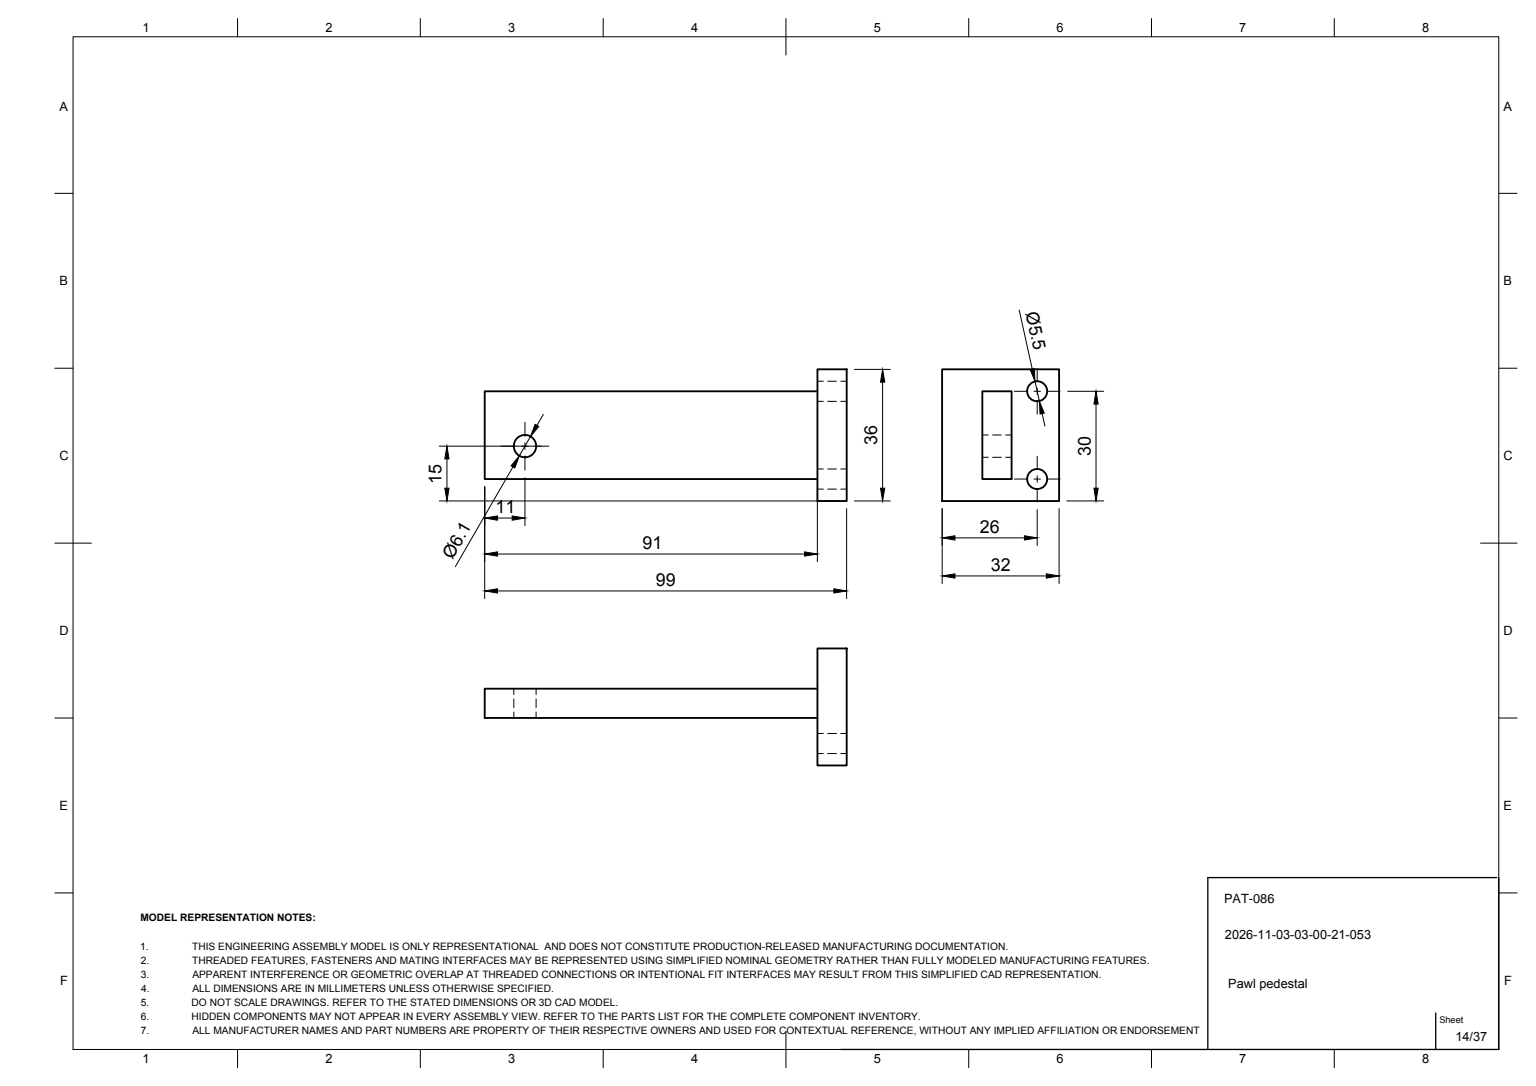
ISO-10303-21;
HEADER;
/* Generated by software containing ST-Developer
 * from STEP Tools, Inc. (www.steptools.com) 
 */

FILE_DESCRIPTION(
/* description */ ('Ratchet and pawl hand winch drum'),
/* implementation_level */ '2;1');

FILE_NAME(
/* name */ 'Pawl pedestal.step',
/* time_stamp */ '2026-10-27T12:42:58-07:00',
/* author */ (''),
/* organization */ (''),
/* preprocessor_version */ 'ST-DEVELOPER v20.2',
/* originating_system */ 'Autodesk Translation Framework v15.17.0.0',
/* authorisation */ '');

FILE_SCHEMA (('AUTOMOTIVE_DESIGN { 1 0 10303 214 3 1 1 }'));
ENDSEC;

DATA;
#10=MECHANICAL_DESIGN_GEOMETRIC_PRESENTATION_REPRESENTATION('',(#398),#11801);
#330=SHAPE_REPRESENTATION_RELATIONSHIP('SRR','None',#11956,#364);
#364=ADVANCED_BREP_SHAPE_REPRESENTATION('',(#433),#11773);
#398=STYLED_ITEM('',(#12206),#433);
#433=MANIFOLD_SOLID_BREP('Body1',#6275);
#516=FACE_BOUND('',#1344,.T.);
#517=FACE_BOUND('',#1345,.T.);
#518=FACE_BOUND('',#1346,.T.);
#519=FACE_BOUND('',#1352,.T.);
#520=FACE_BOUND('',#1355,.T.);
#521=FACE_BOUND('',#1359,.T.);
#522=FACE_BOUND('',#1360,.T.);
#647=PLANE('',#6860);
#648=PLANE('',#6861);
#649=PLANE('',#6862);
#650=PLANE('',#6863);
#651=PLANE('',#6864);
#652=PLANE('',#6865);
#653=PLANE('',#6866);
#654=PLANE('',#6867);
#655=PLANE('',#6868);
#656=PLANE('',#6869);
#657=PLANE('',#6870);
#924=FACE_OUTER_BOUND('',#1340,.T.);
#925=FACE_OUTER_BOUND('',#1341,.T.);
#926=FACE_OUTER_BOUND('',#1342,.T.);
#927=FACE_OUTER_BOUND('',#1343,.T.);
#928=FACE_OUTER_BOUND('',#1347,.T.);
#929=FACE_OUTER_BOUND('',#1348,.T.);
#930=FACE_OUTER_BOUND('',#1349,.T.);
#931=FACE_OUTER_BOUND('',#1350,.T.);
#932=FACE_OUTER_BOUND('',#1351,.T.);
#933=FACE_OUTER_BOUND('',#1353,.T.);
#934=FACE_OUTER_BOUND('',#1354,.T.);
#935=FACE_OUTER_BOUND('',#1356,.T.);
#936=FACE_OUTER_BOUND('',#1357,.T.);
#937=FACE_OUTER_BOUND('',#1358,.T.);
#1340=EDGE_LOOP('',(#4595,#4596,#4597,#4598));
#1341=EDGE_LOOP('',(#4599,#4600,#4601,#4602));
#1342=EDGE_LOOP('',(#4603,#4604,#4605,#4606));
#1343=EDGE_LOOP('',(#4607,#4608,#4609,#4610));
#1344=EDGE_LOOP('',(#4611));
#1345=EDGE_LOOP('',(#4612));
#1346=EDGE_LOOP('',(#4613,#4614,#4615,#4616));
#1347=EDGE_LOOP('',(#4617,#4618,#4619,#4620));
#1348=EDGE_LOOP('',(#4621,#4622,#4623,#4624));
#1349=EDGE_LOOP('',(#4625,#4626,#4627,#4628));
#1350=EDGE_LOOP('',(#4629,#4630,#4631,#4632));
#1351=EDGE_LOOP('',(#4633,#4634,#4635,#4636));
#1352=EDGE_LOOP('',(#4637));
#1353=EDGE_LOOP('',(#4638,#4639,#4640,#4641));
#1354=EDGE_LOOP('',(#4642,#4643,#4644,#4645));
#1355=EDGE_LOOP('',(#4646));
#1356=EDGE_LOOP('',(#4647,#4648,#4649,#4650));
#1357=EDGE_LOOP('',(#4651,#4652,#4653,#4654));
#1358=EDGE_LOOP('',(#4655,#4656,#4657,#4658));
#1359=EDGE_LOOP('',(#4659));
#1360=EDGE_LOOP('',(#4660));
#1795=LINE('',#9617,#2306);
#1796=LINE('',#9623,#2307);
#1797=LINE('',#9629,#2308);
#1798=LINE('',#9634,#2309);
#1799=LINE('',#9636,#2310);
#1800=LINE('',#9638,#2311);
#1801=LINE('',#9639,#2312);
#1802=LINE('',#9642,#2313);
#1803=LINE('',#9644,#2314);
#1804=LINE('',#9646,#2315);
#1805=LINE('',#9647,#2316);
#1806=LINE('',#9650,#2317);
#1807=LINE('',#9652,#2318);
#1808=LINE('',#9653,#2319);
#1809=LINE('',#9656,#2320);
#1810=LINE('',#9658,#2321);
#1811=LINE('',#9659,#2322);
#1812=LINE('',#9661,#2323);
#1813=LINE('',#9663,#2324);
#1814=LINE('',#9666,#2325);
#1815=LINE('',#9668,#2326);
#1816=LINE('',#9669,#2327);
#1817=LINE('',#9672,#2328);
#1818=LINE('',#9673,#2329);
#1819=LINE('',#9676,#2330);
#1820=LINE('',#9677,#2331);
#1821=LINE('',#9679,#2332);
#2306=VECTOR('',#7804,0.275);
#2307=VECTOR('',#7811,0.275);
#2308=VECTOR('',#7818,0.305);
#2309=VECTOR('',#7823,1.);
#2310=VECTOR('',#7824,1.);
#2311=VECTOR('',#7825,1.);
#2312=VECTOR('',#7826,1.);
#2313=VECTOR('',#7827,1.);
#2314=VECTOR('',#7828,1.);
#2315=VECTOR('',#7829,1.);
#2316=VECTOR('',#7830,1.);
#2317=VECTOR('',#7833,1.);
#2318=VECTOR('',#7834,1.);
#2319=VECTOR('',#7835,1.);
#2320=VECTOR('',#7838,1.);
#2321=VECTOR('',#7839,1.);
#2322=VECTOR('',#7840,1.);
#2323=VECTOR('',#7843,1.);
#2324=VECTOR('',#7846,1.);
#2325=VECTOR('',#7849,1.);
#2326=VECTOR('',#7850,1.);
#2327=VECTOR('',#7851,1.);
#2328=VECTOR('',#7854,1.);
#2329=VECTOR('',#7855,1.);
#2330=VECTOR('',#7858,1.);
#2331=VECTOR('',#7859,1.);
#2332=VECTOR('',#7862,1.);
#2795=CIRCLE('',#6852,0.275);
#2796=CIRCLE('',#6853,0.275);
#2797=CIRCLE('',#6855,0.275);
#2798=CIRCLE('',#6856,0.275);
#2799=CIRCLE('',#6858,0.305);
#2800=CIRCLE('',#6859,0.305);
#3058=VERTEX_POINT('',#9614);
#3059=VERTEX_POINT('',#9616);
#3060=VERTEX_POINT('',#9620);
#3061=VERTEX_POINT('',#9622);
#3062=VERTEX_POINT('',#9626);
#3063=VERTEX_POINT('',#9628);
#3064=VERTEX_POINT('',#9632);
#3065=VERTEX_POINT('',#9633);
#3066=VERTEX_POINT('',#9635);
#3067=VERTEX_POINT('',#9637);
#3068=VERTEX_POINT('',#9640);
#3069=VERTEX_POINT('',#9641);
#3070=VERTEX_POINT('',#9643);
#3071=VERTEX_POINT('',#9645);
#3072=VERTEX_POINT('',#9649);
#3073=VERTEX_POINT('',#9651);
#3074=VERTEX_POINT('',#9655);
#3075=VERTEX_POINT('',#9657);
#3076=VERTEX_POINT('',#9665);
#3077=VERTEX_POINT('',#9667);
#3078=VERTEX_POINT('',#9671);
#3079=VERTEX_POINT('',#9675);
#3641=EDGE_CURVE('',#3058,#3058,#2795,.T.);
#3642=EDGE_CURVE('',#3058,#3059,#1795,.T.);
#3643=EDGE_CURVE('',#3059,#3059,#2796,.T.);
#3644=EDGE_CURVE('',#3060,#3060,#2797,.T.);
#3645=EDGE_CURVE('',#3060,#3061,#1796,.T.);
#3646=EDGE_CURVE('',#3061,#3061,#2798,.T.);
#3647=EDGE_CURVE('',#3062,#3062,#2799,.T.);
#3648=EDGE_CURVE('',#3062,#3063,#1797,.T.);
#3649=EDGE_CURVE('',#3063,#3063,#2800,.T.);
#3650=EDGE_CURVE('',#3064,#3065,#1798,.T.);
#3651=EDGE_CURVE('',#3064,#3066,#1799,.T.);
#3652=EDGE_CURVE('',#3067,#3066,#1800,.T.);
#3653=EDGE_CURVE('',#3065,#3067,#1801,.T.);
#3654=EDGE_CURVE('',#3068,#3069,#1802,.T.);
#3655=EDGE_CURVE('',#3070,#3068,#1803,.T.);
#3656=EDGE_CURVE('',#3071,#3070,#1804,.T.);
#3657=EDGE_CURVE('',#3069,#3071,#1805,.T.);
#3658=EDGE_CURVE('',#3065,#3072,#1806,.T.);
#3659=EDGE_CURVE('',#3073,#3067,#1807,.T.);
#3660=EDGE_CURVE('',#3072,#3073,#1808,.T.);
#3661=EDGE_CURVE('',#3074,#3064,#1809,.T.);
#3662=EDGE_CURVE('',#3074,#3075,#1810,.T.);
#3663=EDGE_CURVE('',#3066,#3075,#1811,.T.);
#3664=EDGE_CURVE('',#3075,#3073,#1812,.T.);
#3665=EDGE_CURVE('',#3072,#3074,#1813,.T.);
#3666=EDGE_CURVE('',#3070,#3076,#1814,.T.);
#3667=EDGE_CURVE('',#3077,#3076,#1815,.T.);
#3668=EDGE_CURVE('',#3071,#3077,#1816,.T.);
#3669=EDGE_CURVE('',#3068,#3078,#1817,.T.);
#3670=EDGE_CURVE('',#3076,#3078,#1818,.T.);
#3671=EDGE_CURVE('',#3069,#3079,#1819,.T.);
#3672=EDGE_CURVE('',#3078,#3079,#1820,.T.);
#3673=EDGE_CURVE('',#3079,#3077,#1821,.T.);
#4595=ORIENTED_EDGE('',*,*,#3641,.F.);
#4596=ORIENTED_EDGE('',*,*,#3642,.T.);
#4597=ORIENTED_EDGE('',*,*,#3643,.F.);
#4598=ORIENTED_EDGE('',*,*,#3642,.F.);
#4599=ORIENTED_EDGE('',*,*,#3644,.F.);
#4600=ORIENTED_EDGE('',*,*,#3645,.T.);
#4601=ORIENTED_EDGE('',*,*,#3646,.F.);
#4602=ORIENTED_EDGE('',*,*,#3645,.F.);
#4603=ORIENTED_EDGE('',*,*,#3647,.F.);
#4604=ORIENTED_EDGE('',*,*,#3648,.T.);
#4605=ORIENTED_EDGE('',*,*,#3649,.F.);
#4606=ORIENTED_EDGE('',*,*,#3648,.F.);
#4607=ORIENTED_EDGE('',*,*,#3650,.F.);
#4608=ORIENTED_EDGE('',*,*,#3651,.T.);
#4609=ORIENTED_EDGE('',*,*,#3652,.F.);
#4610=ORIENTED_EDGE('',*,*,#3653,.F.);
#4611=ORIENTED_EDGE('',*,*,#3643,.T.);
#4612=ORIENTED_EDGE('',*,*,#3646,.T.);
#4613=ORIENTED_EDGE('',*,*,#3654,.F.);
#4614=ORIENTED_EDGE('',*,*,#3655,.F.);
#4615=ORIENTED_EDGE('',*,*,#3656,.F.);
#4616=ORIENTED_EDGE('',*,*,#3657,.F.);
#4617=ORIENTED_EDGE('',*,*,#3658,.F.);
#4618=ORIENTED_EDGE('',*,*,#3653,.T.);
#4619=ORIENTED_EDGE('',*,*,#3659,.F.);
#4620=ORIENTED_EDGE('',*,*,#3660,.F.);
#4621=ORIENTED_EDGE('',*,*,#3661,.F.);
#4622=ORIENTED_EDGE('',*,*,#3662,.T.);
#4623=ORIENTED_EDGE('',*,*,#3663,.F.);
#4624=ORIENTED_EDGE('',*,*,#3651,.F.);
#4625=ORIENTED_EDGE('',*,*,#3652,.T.);
#4626=ORIENTED_EDGE('',*,*,#3663,.T.);
#4627=ORIENTED_EDGE('',*,*,#3664,.T.);
#4628=ORIENTED_EDGE('',*,*,#3659,.T.);
#4629=ORIENTED_EDGE('',*,*,#3650,.T.);
#4630=ORIENTED_EDGE('',*,*,#3658,.T.);
#4631=ORIENTED_EDGE('',*,*,#3665,.T.);
#4632=ORIENTED_EDGE('',*,*,#3661,.T.);
#4633=ORIENTED_EDGE('',*,*,#3656,.T.);
#4634=ORIENTED_EDGE('',*,*,#3666,.T.);
#4635=ORIENTED_EDGE('',*,*,#3667,.F.);
#4636=ORIENTED_EDGE('',*,*,#3668,.F.);
#4637=ORIENTED_EDGE('',*,*,#3647,.T.);
#4638=ORIENTED_EDGE('',*,*,#3655,.T.);
#4639=ORIENTED_EDGE('',*,*,#3669,.T.);
#4640=ORIENTED_EDGE('',*,*,#3670,.F.);
#4641=ORIENTED_EDGE('',*,*,#3666,.F.);
#4642=ORIENTED_EDGE('',*,*,#3654,.T.);
#4643=ORIENTED_EDGE('',*,*,#3671,.T.);
#4644=ORIENTED_EDGE('',*,*,#3672,.F.);
#4645=ORIENTED_EDGE('',*,*,#3669,.F.);
#4646=ORIENTED_EDGE('',*,*,#3649,.T.);
#4647=ORIENTED_EDGE('',*,*,#3657,.T.);
#4648=ORIENTED_EDGE('',*,*,#3668,.T.);
#4649=ORIENTED_EDGE('',*,*,#3673,.F.);
#4650=ORIENTED_EDGE('',*,*,#3671,.F.);
#4651=ORIENTED_EDGE('',*,*,#3673,.T.);
#4652=ORIENTED_EDGE('',*,*,#3667,.T.);
#4653=ORIENTED_EDGE('',*,*,#3670,.T.);
#4654=ORIENTED_EDGE('',*,*,#3672,.T.);
#4655=ORIENTED_EDGE('',*,*,#3665,.F.);
#4656=ORIENTED_EDGE('',*,*,#3660,.T.);
#4657=ORIENTED_EDGE('',*,*,#3664,.F.);
#4658=ORIENTED_EDGE('',*,*,#3662,.F.);
#4659=ORIENTED_EDGE('',*,*,#3641,.T.);
#4660=ORIENTED_EDGE('',*,*,#3644,.T.);
#5845=CYLINDRICAL_SURFACE('',#6851,0.275);
#5846=CYLINDRICAL_SURFACE('',#6854,0.275);
#5847=CYLINDRICAL_SURFACE('',#6857,0.305);
#5994=ADVANCED_FACE('',(#924),#5845,.F.);
#5995=ADVANCED_FACE('',(#925),#5846,.F.);
#5996=ADVANCED_FACE('',(#926),#5847,.F.);
#5997=ADVANCED_FACE('',(#927,#516,#517,#518),#647,.T.);
#5998=ADVANCED_FACE('',(#928),#648,.T.);
#5999=ADVANCED_FACE('',(#929),#649,.T.);
#6000=ADVANCED_FACE('',(#930),#650,.T.);
#6001=ADVANCED_FACE('',(#931),#651,.F.);
#6002=ADVANCED_FACE('',(#932,#519),#652,.T.);
#6003=ADVANCED_FACE('',(#933),#653,.T.);
#6004=ADVANCED_FACE('',(#934,#520),#654,.T.);
#6005=ADVANCED_FACE('',(#935),#655,.T.);
#6006=ADVANCED_FACE('',(#936),#656,.T.);
#6007=ADVANCED_FACE('',(#937,#521,#522),#657,.F.);
#6275=CLOSED_SHELL('',(#5994,#5995,#5996,#5997,#5998,#5999,#6000,#6001,
#6002,#6003,#6004,#6005,#6006,#6007));
#6850=AXIS2_PLACEMENT_3D('',#9612,#7798,#7799);
#6851=AXIS2_PLACEMENT_3D('',#9613,#7800,#7801);
#6852=AXIS2_PLACEMENT_3D('',#9615,#7802,#7803);
#6853=AXIS2_PLACEMENT_3D('',#9618,#7805,#7806);
#6854=AXIS2_PLACEMENT_3D('',#9619,#7807,#7808);
#6855=AXIS2_PLACEMENT_3D('',#9621,#7809,#7810);
#6856=AXIS2_PLACEMENT_3D('',#9624,#7812,#7813);
#6857=AXIS2_PLACEMENT_3D('',#9625,#7814,#7815);
#6858=AXIS2_PLACEMENT_3D('',#9627,#7816,#7817);
#6859=AXIS2_PLACEMENT_3D('',#9630,#7819,#7820);
#6860=AXIS2_PLACEMENT_3D('',#9631,#7821,#7822);
#6861=AXIS2_PLACEMENT_3D('',#9648,#7831,#7832);
#6862=AXIS2_PLACEMENT_3D('',#9654,#7836,#7837);
#6863=AXIS2_PLACEMENT_3D('',#9660,#7841,#7842);
#6864=AXIS2_PLACEMENT_3D('',#9662,#7844,#7845);
#6865=AXIS2_PLACEMENT_3D('',#9664,#7847,#7848);
#6866=AXIS2_PLACEMENT_3D('',#9670,#7852,#7853);
#6867=AXIS2_PLACEMENT_3D('',#9674,#7856,#7857);
#6868=AXIS2_PLACEMENT_3D('',#9678,#7860,#7861);
#6869=AXIS2_PLACEMENT_3D('',#9680,#7863,#7864);
#6870=AXIS2_PLACEMENT_3D('',#9681,#7865,#7866);
#7798=DIRECTION('axis',(0.,0.,1.));
#7799=DIRECTION('refdir',(1.,0.,0.));
#7800=DIRECTION('center_axis',(0.,0.,1.));
#7801=DIRECTION('ref_axis',(1.,0.,0.));
#7802=DIRECTION('center_axis',(0.,0.,1.));
#7803=DIRECTION('ref_axis',(1.,0.,0.));
#7804=DIRECTION('',(0.,0.,1.));
#7805=DIRECTION('center_axis',(0.,0.,-1.));
#7806=DIRECTION('ref_axis',(1.,0.,0.));
#7807=DIRECTION('center_axis',(0.,0.,1.));
#7808=DIRECTION('ref_axis',(1.,0.,0.));
#7809=DIRECTION('center_axis',(0.,0.,1.));
#7810=DIRECTION('ref_axis',(1.,0.,0.));
#7811=DIRECTION('',(0.,0.,1.));
#7812=DIRECTION('center_axis',(0.,0.,-1.));
#7813=DIRECTION('ref_axis',(1.,0.,0.));
#7814=DIRECTION('center_axis',(0.,1.,0.));
#7815=DIRECTION('ref_axis',(1.,0.,0.));
#7816=DIRECTION('center_axis',(0.,1.,0.));
#7817=DIRECTION('ref_axis',(1.,0.,0.));
#7818=DIRECTION('',(0.,1.,0.));
#7819=DIRECTION('center_axis',(0.,-1.,0.));
#7820=DIRECTION('ref_axis',(1.,0.,0.));
#7821=DIRECTION('center_axis',(0.,0.,1.));
#7822=DIRECTION('ref_axis',(1.,0.,0.));
#7823=DIRECTION('',(-1.,0.,0.));
#7824=DIRECTION('',(0.,1.,0.));
#7825=DIRECTION('',(1.,0.,0.));
#7826=DIRECTION('',(0.,1.,0.));
#7827=DIRECTION('',(-1.,0.,0.));
#7828=DIRECTION('',(0.,1.,0.));
#7829=DIRECTION('',(1.,0.,0.));
#7830=DIRECTION('',(0.,-1.,0.));
#7831=DIRECTION('center_axis',(-1.,0.,0.));
#7832=DIRECTION('ref_axis',(0.,0.,1.));
#7833=DIRECTION('',(0.,0.,-1.));
#7834=DIRECTION('',(0.,0.,1.));
#7835=DIRECTION('',(0.,1.,0.));
#7836=DIRECTION('center_axis',(1.,0.,0.));
#7837=DIRECTION('ref_axis',(0.,0.,-1.));
#7838=DIRECTION('',(0.,0.,1.));
#7839=DIRECTION('',(0.,1.,0.));
#7840=DIRECTION('',(0.,0.,-1.));
#7841=DIRECTION('center_axis',(0.,1.,0.));
#7842=DIRECTION('ref_axis',(0.,0.,1.));
#7843=DIRECTION('',(-1.,0.,0.));
#7844=DIRECTION('center_axis',(0.,1.,0.));
#7845=DIRECTION('ref_axis',(1.,0.,0.));
#7846=DIRECTION('',(1.,0.,0.));
#7847=DIRECTION('center_axis',(0.,-1.,0.));
#7848=DIRECTION('ref_axis',(1.,0.,0.));
#7849=DIRECTION('',(0.,0.,1.));
#7850=DIRECTION('',(1.,0.,0.));
#7851=DIRECTION('',(0.,0.,1.));
#7852=DIRECTION('center_axis',(1.,0.,0.));
#7853=DIRECTION('ref_axis',(0.,1.,0.));
#7854=DIRECTION('',(0.,0.,1.));
#7855=DIRECTION('',(0.,1.,0.));
#7856=DIRECTION('center_axis',(0.,1.,0.));
#7857=DIRECTION('ref_axis',(-1.,0.,0.));
#7858=DIRECTION('',(0.,0.,1.));
#7859=DIRECTION('',(-1.,0.,0.));
#7860=DIRECTION('center_axis',(-1.,0.,0.));
#7861=DIRECTION('ref_axis',(0.,-1.,0.));
#7862=DIRECTION('',(0.,-1.,0.));
#7863=DIRECTION('center_axis',(0.,0.,1.));
#7864=DIRECTION('ref_axis',(1.,0.,0.));
#7865=DIRECTION('center_axis',(0.,0.,1.));
#7866=DIRECTION('ref_axis',(1.,0.,0.));
#9612=CARTESIAN_POINT('',(0.,0.,0.));
#9613=CARTESIAN_POINT('Origin',(8.,-5.9,1.1));
#9614=CARTESIAN_POINT('',(7.725,-5.9,1.2));
#9615=CARTESIAN_POINT('Origin',(8.,-5.9,1.2));
#9616=CARTESIAN_POINT('',(7.725,-5.9,2.));
#9617=CARTESIAN_POINT('',(7.725,-5.9,1.1));
#9618=CARTESIAN_POINT('Origin',(8.,-5.9,2.));
#9619=CARTESIAN_POINT('Origin',(5.6,-5.9,1.1));
#9620=CARTESIAN_POINT('',(5.325,-5.9,1.2));
#9621=CARTESIAN_POINT('Origin',(5.6,-5.9,1.2));
#9622=CARTESIAN_POINT('',(5.325,-5.9,2.));
#9623=CARTESIAN_POINT('',(5.325,-5.9,1.1));
#9624=CARTESIAN_POINT('Origin',(5.6,-5.9,2.));
#9625=CARTESIAN_POINT('Origin',(6.5,-5.3,10.));
#9626=CARTESIAN_POINT('',(6.195,-5.2,10.));
#9627=CARTESIAN_POINT('Origin',(6.5,-5.2,10.));
#9628=CARTESIAN_POINT('',(6.195,-4.4,10.));
#9629=CARTESIAN_POINT('',(6.195,-5.3,10.));
#9630=CARTESIAN_POINT('Origin',(6.5,-4.4,10.));
#9631=CARTESIAN_POINT('Origin',(5.,-6.5,2.));
#9632=CARTESIAN_POINT('',(8.6,-6.5,2.));
#9633=CARTESIAN_POINT('',(5.,-6.5,2.));
#9634=CARTESIAN_POINT('',(8.6,-6.5,2.));
#9635=CARTESIAN_POINT('',(8.6,-3.3,2.));
#9636=CARTESIAN_POINT('',(8.6,-6.5,2.));
#9637=CARTESIAN_POINT('',(5.,-3.3,2.));
#9638=CARTESIAN_POINT('',(8.6,-3.3,2.));
#9639=CARTESIAN_POINT('',(5.,-6.5,2.));
#9640=CARTESIAN_POINT('',(8.,-4.4,2.));
#9641=CARTESIAN_POINT('',(5.6,-4.4,2.));
#9642=CARTESIAN_POINT('',(6.5,-4.4,2.));
#9643=CARTESIAN_POINT('',(8.,-5.2,2.));
#9644=CARTESIAN_POINT('',(8.,-5.85,2.));
#9645=CARTESIAN_POINT('',(5.6,-5.2,2.));
#9646=CARTESIAN_POINT('',(5.3,-5.2,2.));
#9647=CARTESIAN_POINT('',(5.6,-5.45,2.));
#9648=CARTESIAN_POINT('Origin',(5.,-6.5,1.2));
#9649=CARTESIAN_POINT('',(5.,-6.5,1.2));
#9650=CARTESIAN_POINT('',(5.,-6.5,2.));
#9651=CARTESIAN_POINT('',(5.,-3.3,1.2));
#9652=CARTESIAN_POINT('',(5.,-3.3,2.));
#9653=CARTESIAN_POINT('',(5.,-6.5,1.2));
#9654=CARTESIAN_POINT('Origin',(8.6,-6.5,2.));
#9655=CARTESIAN_POINT('',(8.6,-6.5,1.2));
#9656=CARTESIAN_POINT('',(8.6,-6.5,1.2));
#9657=CARTESIAN_POINT('',(8.6,-3.3,1.2));
#9658=CARTESIAN_POINT('',(8.6,-6.5,1.2));
#9659=CARTESIAN_POINT('',(8.6,-3.3,1.2));
#9660=CARTESIAN_POINT('Origin',(6.8,-3.3,1.6));
#9661=CARTESIAN_POINT('',(5.,-3.3,1.2));
#9662=CARTESIAN_POINT('Origin',(6.8,-6.5,1.6));
#9663=CARTESIAN_POINT('',(5.,-6.5,1.2));
#9664=CARTESIAN_POINT('Origin',(5.6,-5.2,1.2));
#9665=CARTESIAN_POINT('',(8.,-5.2,11.1));
#9666=CARTESIAN_POINT('',(8.,-5.2,1.2));
#9667=CARTESIAN_POINT('',(5.6,-5.2,11.1));
#9668=CARTESIAN_POINT('',(5.6,-5.2,11.1));
#9669=CARTESIAN_POINT('',(5.6,-5.2,1.2));
#9670=CARTESIAN_POINT('Origin',(8.,-5.2,1.2));
#9671=CARTESIAN_POINT('',(8.,-4.4,11.1));
#9672=CARTESIAN_POINT('',(8.,-4.4,1.2));
#9673=CARTESIAN_POINT('',(8.,-5.2,11.1));
#9674=CARTESIAN_POINT('Origin',(8.,-4.4,1.2));
#9675=CARTESIAN_POINT('',(5.6,-4.4,11.1));
#9676=CARTESIAN_POINT('',(5.6,-4.4,1.2));
#9677=CARTESIAN_POINT('',(8.,-4.4,11.1));
#9678=CARTESIAN_POINT('Origin',(5.6,-4.4,1.2));
#9679=CARTESIAN_POINT('',(5.6,-4.4,11.1));
#9680=CARTESIAN_POINT('Origin',(6.8,-4.8,11.1));
#9681=CARTESIAN_POINT('Origin',(6.8,-4.8,1.2));
#11733=UNCERTAINTY_MEASURE_WITH_UNIT(LENGTH_MEASURE(0.001),#11802,
'DISTANCE_ACCURACY_VALUE',
'Maximum model space distance between geometric entities at asserted c
onnectivities');
#11761=UNCERTAINTY_MEASURE_WITH_UNIT(LENGTH_MEASURE(0.001),#11802,
'DISTANCE_ACCURACY_VALUE',
'Maximum model space distance between geometric entities at asserted c
onnectivities');
#11773=(
GEOMETRIC_REPRESENTATION_CONTEXT(3)
GLOBAL_UNCERTAINTY_ASSIGNED_CONTEXT((#11733))
GLOBAL_UNIT_ASSIGNED_CONTEXT((#11802,#11804,#11805))
REPRESENTATION_CONTEXT('','3D')
);
#11801=(
GEOMETRIC_REPRESENTATION_CONTEXT(3)
GLOBAL_UNCERTAINTY_ASSIGNED_CONTEXT((#11761))
GLOBAL_UNIT_ASSIGNED_CONTEXT((#11802,#11804,#11805))
REPRESENTATION_CONTEXT('','3D')
);
#11802=(
LENGTH_UNIT()
NAMED_UNIT(*)
SI_UNIT(.CENTI.,.METRE.)
);
#11804=(
NAMED_UNIT(*)
PLANE_ANGLE_UNIT()
SI_UNIT($,.RADIAN.)
);
#11805=(
NAMED_UNIT(*)
SI_UNIT($,.STERADIAN.)
SOLID_ANGLE_UNIT()
);
#11817=SHAPE_DEFINITION_REPRESENTATION(#11856,#11956);
#11856=PRODUCT_DEFINITION_SHAPE('',$,#11996);
#11956=SHAPE_REPRESENTATION('',(#6850),#11773);
#11984=PRODUCT_DEFINITION_CONTEXT('part definition',#12103,'design');
#11996=PRODUCT_DEFINITION('Pawl pedestal','Pawl pedestal',#12035,#11984);
#12035=PRODUCT_DEFINITION_FORMATION('',$,#12116);
#12103=APPLICATION_CONTEXT(
'Core Data for Automotive Mechanical Design Process');
#12104=PRODUCT_CONTEXT('part definition',#12103,'mechanical');
#12116=PRODUCT('Pawl pedestal','Pawl pedestal','Pawl pedestal',(#12104));
#12200=COLOUR_RGB('Sky Blue',0.24,0.69,0.87);
#12201=FILL_AREA_STYLE_COLOUR('',#12200);
#12202=FILL_AREA_STYLE('',(#12201));
#12203=SURFACE_STYLE_FILL_AREA(#12202);
#12204=SURFACE_SIDE_STYLE('',(#12203));
#12205=SURFACE_STYLE_USAGE(.BOTH.,#12204);
#12206=PRESENTATION_STYLE_ASSIGNMENT((#12205));
ENDSEC;
END-ISO-10303-21;
